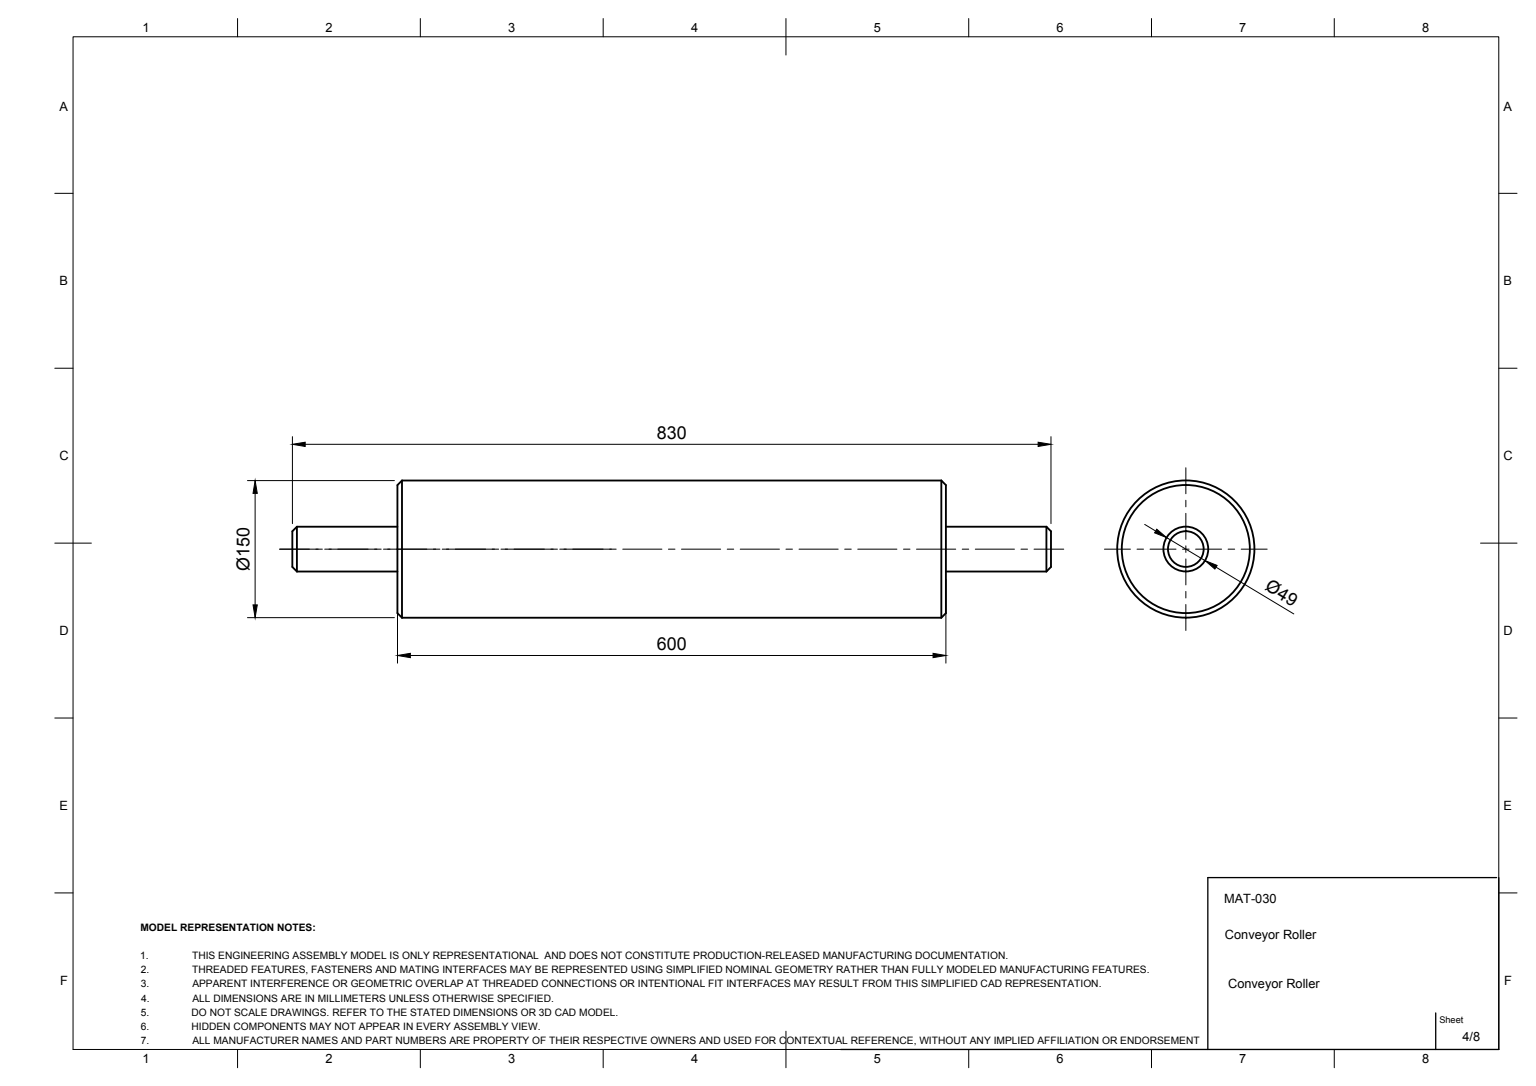
ISO-10303-21;
HEADER;
/* Generated by software containing ST-Developer
 * from STEP Tools, Inc. (www.steptools.com) 
 */

FILE_DESCRIPTION(
/* description */ ('STEP AP214'),
/* implementation_level */ '2;1');

FILE_NAME(
/* name */ 'Conveyor Roller.step',
/* time_stamp */ '2026-11-14T06:43:04-08:00',
/* author */ (''),
/* organization */ (''),
/* preprocessor_version */ 'ST-DEVELOPER v20.2',
/* originating_system */ 'Autodesk Translation Framework v15.17.0.0',
/* authorisation */ '');

FILE_SCHEMA (('AUTOMOTIVE_DESIGN { 1 0 10303 214 3 1 1 }'));
ENDSEC;

DATA;
#10=MECHANICAL_DESIGN_GEOMETRIC_PRESENTATION_REPRESENTATION('',(#205),#5658);
#107=CONICAL_SURFACE('',#3433,70.0000000000001,0.785398163397444);
#108=CONICAL_SURFACE('',#3437,19.5,0.785398163397451);
#109=CONICAL_SURFACE('',#3441,24.5,0.78539816339745);
#110=CONICAL_SURFACE('',#3444,75.,0.785398163397444);
#183=SHAPE_REPRESENTATION_RELATIONSHIP('SRR','None',#5713,#194);
#194=ADVANCED_BREP_SHAPE_REPRESENTATION('',(#216),#5654);
#205=STYLED_ITEM('',(#5773),#216);
#216=MANIFOLD_SOLID_BREP('Body1',#3067);
#262=CYLINDRICAL_SURFACE('',#3447,75.);
#263=CYLINDRICAL_SURFACE('',#3448,24.5);
#264=CYLINDRICAL_SURFACE('',#3450,24.5);
#329=FACE_BOUND('',#711,.T.);
#330=FACE_BOUND('',#713,.T.);
#462=FACE_OUTER_BOUND('',#702,.T.);
#463=FACE_OUTER_BOUND('',#703,.T.);
#464=FACE_OUTER_BOUND('',#704,.T.);
#465=FACE_OUTER_BOUND('',#705,.T.);
#466=FACE_OUTER_BOUND('',#706,.T.);
#467=FACE_OUTER_BOUND('',#707,.T.);
#468=FACE_OUTER_BOUND('',#708,.T.);
#469=FACE_OUTER_BOUND('',#709,.T.);
#470=FACE_OUTER_BOUND('',#710,.T.);
#471=FACE_OUTER_BOUND('',#712,.T.);
#472=FACE_OUTER_BOUND('',#714,.T.);
#702=EDGE_LOOP('',(#2556,#2557,#2558,#2559,#2560));
#703=EDGE_LOOP('',(#2561,#2562,#2563,#2564,#2565));
#704=EDGE_LOOP('',(#2566,#2567,#2568,#2569));
#705=EDGE_LOOP('',(#2570,#2571,#2572,#2573));
#706=EDGE_LOOP('',(#2574,#2575,#2576,#2577,#2578));
#707=EDGE_LOOP('',(#2579,#2580,#2581,#2582));
#708=EDGE_LOOP('',(#2583,#2584,#2585,#2586,#2587));
#709=EDGE_LOOP('',(#2588));
#710=EDGE_LOOP('',(#2589));
#711=EDGE_LOOP('',(#2590));
#712=EDGE_LOOP('',(#2591));
#713=EDGE_LOOP('',(#2592));
#714=EDGE_LOOP('',(#2593));
#896=LINE('',#5374,#1092);
#897=LINE('',#5382,#1093);
#898=LINE('',#5388,#1094);
#899=LINE('',#5394,#1095);
#900=LINE('',#5397,#1096);
#901=LINE('',#5401,#1097);
#902=LINE('',#5404,#1098);
#1092=VECTOR('',#4174,70.0000000000001);
#1093=VECTOR('',#4183,19.5);
#1094=VECTOR('',#4190,24.5);
#1095=VECTOR('',#4197,75.);
#1096=VECTOR('',#4202,75.);
#1097=VECTOR('',#4207,24.5);
#1098=VECTOR('',#4210,24.5);
#1266=CIRCLE('',#3434,75.);
#1267=CIRCLE('',#3435,75.);
#1268=CIRCLE('',#3436,70.0000000000001);
#1269=CIRCLE('',#3438,24.5);
#1270=CIRCLE('',#3439,24.5);
#1271=CIRCLE('',#3440,19.5);
#1272=CIRCLE('',#3442,24.5);
#1273=CIRCLE('',#3443,19.5);
#1274=CIRCLE('',#3445,75.);
#1275=CIRCLE('',#3446,70.);
#1276=CIRCLE('',#3449,24.5);
#1277=CIRCLE('',#3451,24.5);
#1499=VERTEX_POINT('',#5369);
#1500=VERTEX_POINT('',#5370);
#1501=VERTEX_POINT('',#5373);
#1502=VERTEX_POINT('',#5377);
#1503=VERTEX_POINT('',#5378);
#1504=VERTEX_POINT('',#5381);
#1505=VERTEX_POINT('',#5385);
#1506=VERTEX_POINT('',#5387);
#1507=VERTEX_POINT('',#5391);
#1508=VERTEX_POINT('',#5393);
#1509=VERTEX_POINT('',#5399);
#1510=VERTEX_POINT('',#5403);
#1861=EDGE_CURVE('',#1499,#1500,#1266,.T.);
#1862=EDGE_CURVE('',#1500,#1499,#1267,.T.);
#1863=EDGE_CURVE('',#1500,#1501,#896,.T.);
#1864=EDGE_CURVE('',#1501,#1501,#1268,.T.);
#1865=EDGE_CURVE('',#1502,#1503,#1269,.T.);
#1866=EDGE_CURVE('',#1503,#1502,#1270,.T.);
#1867=EDGE_CURVE('',#1503,#1504,#897,.T.);
#1868=EDGE_CURVE('',#1504,#1504,#1271,.T.);
#1869=EDGE_CURVE('',#1505,#1505,#1272,.T.);
#1870=EDGE_CURVE('',#1505,#1506,#898,.T.);
#1871=EDGE_CURVE('',#1506,#1506,#1273,.T.);
#1872=EDGE_CURVE('',#1507,#1507,#1274,.T.);
#1873=EDGE_CURVE('',#1507,#1508,#899,.T.);
#1874=EDGE_CURVE('',#1508,#1508,#1275,.T.);
#1875=EDGE_CURVE('',#1499,#1507,#900,.T.);
#1876=EDGE_CURVE('',#1509,#1509,#1276,.T.);
#1877=EDGE_CURVE('',#1509,#1505,#901,.T.);
#1878=EDGE_CURVE('',#1502,#1510,#902,.T.);
#1879=EDGE_CURVE('',#1510,#1510,#1277,.T.);
#2556=ORIENTED_EDGE('',*,*,#1861,.F.);
#2557=ORIENTED_EDGE('',*,*,#1862,.F.);
#2558=ORIENTED_EDGE('',*,*,#1863,.T.);
#2559=ORIENTED_EDGE('',*,*,#1864,.F.);
#2560=ORIENTED_EDGE('',*,*,#1863,.F.);
#2561=ORIENTED_EDGE('',*,*,#1865,.F.);
#2562=ORIENTED_EDGE('',*,*,#1866,.F.);
#2563=ORIENTED_EDGE('',*,*,#1867,.T.);
#2564=ORIENTED_EDGE('',*,*,#1868,.F.);
#2565=ORIENTED_EDGE('',*,*,#1867,.F.);
#2566=ORIENTED_EDGE('',*,*,#1869,.F.);
#2567=ORIENTED_EDGE('',*,*,#1870,.T.);
#2568=ORIENTED_EDGE('',*,*,#1871,.F.);
#2569=ORIENTED_EDGE('',*,*,#1870,.F.);
#2570=ORIENTED_EDGE('',*,*,#1872,.F.);
#2571=ORIENTED_EDGE('',*,*,#1873,.T.);
#2572=ORIENTED_EDGE('',*,*,#1874,.F.);
#2573=ORIENTED_EDGE('',*,*,#1873,.F.);
#2574=ORIENTED_EDGE('',*,*,#1861,.T.);
#2575=ORIENTED_EDGE('',*,*,#1862,.T.);
#2576=ORIENTED_EDGE('',*,*,#1875,.T.);
#2577=ORIENTED_EDGE('',*,*,#1872,.T.);
#2578=ORIENTED_EDGE('',*,*,#1875,.F.);
#2579=ORIENTED_EDGE('',*,*,#1876,.F.);
#2580=ORIENTED_EDGE('',*,*,#1877,.T.);
#2581=ORIENTED_EDGE('',*,*,#1869,.T.);
#2582=ORIENTED_EDGE('',*,*,#1877,.F.);
#2583=ORIENTED_EDGE('',*,*,#1865,.T.);
#2584=ORIENTED_EDGE('',*,*,#1866,.T.);
#2585=ORIENTED_EDGE('',*,*,#1878,.T.);
#2586=ORIENTED_EDGE('',*,*,#1879,.T.);
#2587=ORIENTED_EDGE('',*,*,#1878,.F.);
#2588=ORIENTED_EDGE('',*,*,#1871,.T.);
#2589=ORIENTED_EDGE('',*,*,#1874,.T.);
#2590=ORIENTED_EDGE('',*,*,#1876,.T.);
#2591=ORIENTED_EDGE('',*,*,#1864,.T.);
#2592=ORIENTED_EDGE('',*,*,#1879,.F.);
#2593=ORIENTED_EDGE('',*,*,#1868,.T.);
#2842=PLANE('',#3452);
#2843=PLANE('',#3453);
#2844=PLANE('',#3454);
#2845=PLANE('',#3455);
#3003=ADVANCED_FACE('',(#462),#107,.T.);
#3004=ADVANCED_FACE('',(#463),#108,.T.);
#3005=ADVANCED_FACE('',(#464),#109,.T.);
#3006=ADVANCED_FACE('',(#465),#110,.T.);
#3007=ADVANCED_FACE('',(#466),#262,.T.);
#3008=ADVANCED_FACE('',(#467),#263,.T.);
#3009=ADVANCED_FACE('',(#468),#264,.T.);
#3010=ADVANCED_FACE('',(#469),#2842,.T.);
#3011=ADVANCED_FACE('',(#470,#329),#2843,.T.);
#3012=ADVANCED_FACE('',(#471,#330),#2844,.F.);
#3013=ADVANCED_FACE('',(#472),#2845,.F.);
#3067=CLOSED_SHELL('',(#3003,#3004,#3005,#3006,#3007,#3008,#3009,#3010,
#3011,#3012,#3013));
#3432=AXIS2_PLACEMENT_3D('',#5367,#4166,#4167);
#3433=AXIS2_PLACEMENT_3D('',#5368,#4168,#4169);
#3434=AXIS2_PLACEMENT_3D('',#5371,#4170,#4171);
#3435=AXIS2_PLACEMENT_3D('',#5372,#4172,#4173);
#3436=AXIS2_PLACEMENT_3D('',#5375,#4175,#4176);
#3437=AXIS2_PLACEMENT_3D('',#5376,#4177,#4178);
#3438=AXIS2_PLACEMENT_3D('',#5379,#4179,#4180);
#3439=AXIS2_PLACEMENT_3D('',#5380,#4181,#4182);
#3440=AXIS2_PLACEMENT_3D('',#5383,#4184,#4185);
#3441=AXIS2_PLACEMENT_3D('',#5384,#4186,#4187);
#3442=AXIS2_PLACEMENT_3D('',#5386,#4188,#4189);
#3443=AXIS2_PLACEMENT_3D('',#5389,#4191,#4192);
#3444=AXIS2_PLACEMENT_3D('',#5390,#4193,#4194);
#3445=AXIS2_PLACEMENT_3D('',#5392,#4195,#4196);
#3446=AXIS2_PLACEMENT_3D('',#5395,#4198,#4199);
#3447=AXIS2_PLACEMENT_3D('',#5396,#4200,#4201);
#3448=AXIS2_PLACEMENT_3D('',#5398,#4203,#4204);
#3449=AXIS2_PLACEMENT_3D('',#5400,#4205,#4206);
#3450=AXIS2_PLACEMENT_3D('',#5402,#4208,#4209);
#3451=AXIS2_PLACEMENT_3D('',#5405,#4211,#4212);
#3452=AXIS2_PLACEMENT_3D('',#5406,#4213,#4214);
#3453=AXIS2_PLACEMENT_3D('',#5407,#4215,#4216);
#3454=AXIS2_PLACEMENT_3D('',#5408,#4217,#4218);
#3455=AXIS2_PLACEMENT_3D('',#5409,#4219,#4220);
#4166=DIRECTION('axis',(0.,0.,1.));
#4167=DIRECTION('refdir',(1.,0.,0.));
#4168=DIRECTION('center_axis',(0.,-1.,0.));
#4169=DIRECTION('ref_axis',(0.,0.,-1.));
#4170=DIRECTION('center_axis',(0.,-1.,0.));
#4171=DIRECTION('ref_axis',(0.,0.,-1.));
#4172=DIRECTION('center_axis',(0.,-1.,0.));
#4173=DIRECTION('ref_axis',(0.,0.,-1.));
#4174=DIRECTION('',(8.6595605623549E-17,0.70710678118655,-0.707106781186544));
#4175=DIRECTION('center_axis',(0.,1.,0.));
#4176=DIRECTION('ref_axis',(0.,0.,-1.));
#4177=DIRECTION('center_axis',(0.,-1.,0.));
#4178=DIRECTION('ref_axis',(0.,0.,-1.));
#4179=DIRECTION('center_axis',(0.,-1.,0.));
#4180=DIRECTION('ref_axis',(0.,0.,-1.));
#4181=DIRECTION('center_axis',(0.,-1.,0.));
#4182=DIRECTION('ref_axis',(0.,0.,-1.));
#4183=DIRECTION('',(8.65956056235496E-17,0.707106781186546,-0.707106781186549));
#4184=DIRECTION('center_axis',(0.,1.,0.));
#4185=DIRECTION('ref_axis',(0.,0.,-1.));
#4186=DIRECTION('center_axis',(0.,1.,0.));
#4187=DIRECTION('ref_axis',(0.,0.,1.));
#4188=DIRECTION('center_axis',(0.,1.,0.));
#4189=DIRECTION('ref_axis',(0.,0.,-1.));
#4190=DIRECTION('',(8.65956056235495E-17,-0.707106781186546,0.707106781186549));
#4191=DIRECTION('center_axis',(0.,-1.,0.));
#4192=DIRECTION('ref_axis',(0.,0.,-1.));
#4193=DIRECTION('center_axis',(0.,1.,0.));
#4194=DIRECTION('ref_axis',(0.,0.,1.));
#4195=DIRECTION('center_axis',(0.,1.,0.));
#4196=DIRECTION('ref_axis',(0.,0.,-1.));
#4197=DIRECTION('',(8.6595605623549E-17,-0.70710678118655,0.707106781186544));
#4198=DIRECTION('center_axis',(0.,-1.,0.));
#4199=DIRECTION('ref_axis',(0.,0.,-1.));
#4200=DIRECTION('center_axis',(0.,1.,0.));
#4201=DIRECTION('ref_axis',(0.,0.,1.));
#4202=DIRECTION('',(0.,-1.,0.));
#4203=DIRECTION('center_axis',(0.,1.,0.));
#4204=DIRECTION('ref_axis',(0.,0.,1.));
#4205=DIRECTION('center_axis',(0.,1.,0.));
#4206=DIRECTION('ref_axis',(0.,0.,1.));
#4207=DIRECTION('',(0.,-1.,0.));
#4208=DIRECTION('center_axis',(0.,1.,0.));
#4209=DIRECTION('ref_axis',(0.,0.,1.));
#4210=DIRECTION('',(0.,-1.,0.));
#4211=DIRECTION('center_axis',(0.,1.,0.));
#4212=DIRECTION('ref_axis',(0.,0.,1.));
#4213=DIRECTION('center_axis',(0.,-1.,0.));
#4214=DIRECTION('ref_axis',(0.,0.,-1.));
#4215=DIRECTION('center_axis',(0.,-1.,0.));
#4216=DIRECTION('ref_axis',(0.,0.,-1.));
#4217=DIRECTION('center_axis',(0.,-1.,0.));
#4218=DIRECTION('ref_axis',(0.,0.,-1.));
#4219=DIRECTION('center_axis',(0.,-1.,0.));
#4220=DIRECTION('ref_axis',(0.,0.,-1.));
#5367=CARTESIAN_POINT('',(0.,0.,0.));
#5368=CARTESIAN_POINT('Origin',(0.,300.,-2.77555756156289E-14));
#5369=CARTESIAN_POINT('',(9.18485099360515E-15,295.,-75.0000000000001));
#5370=CARTESIAN_POINT('',(-9.18485099360515E-15,295.,75.));
#5371=CARTESIAN_POINT('Origin',(0.,295.,-2.77555756156289E-14));
#5372=CARTESIAN_POINT('Origin',(0.,295.,-2.77555756156289E-14));
#5373=CARTESIAN_POINT('',(-8.57252759403148E-15,300.,70.));
#5374=CARTESIAN_POINT('',(-8.57252759403148E-15,300.,70.));
#5375=CARTESIAN_POINT('Origin',(0.,300.,-2.77555756156289E-14));
#5376=CARTESIAN_POINT('Origin',(0.,415.,-2.77555756156289E-14));
#5377=CARTESIAN_POINT('',(3.00038465791101E-15,410.,-24.5));
#5378=CARTESIAN_POINT('',(-3.00038465791101E-15,410.,24.5));
#5379=CARTESIAN_POINT('Origin',(0.,410.,-2.77555756156289E-14));
#5380=CARTESIAN_POINT('Origin',(0.,410.,-2.77555756156289E-14));
#5381=CARTESIAN_POINT('',(-2.38806125833733E-15,415.,19.4999999999999));
#5382=CARTESIAN_POINT('',(-2.38806125833733E-15,415.,19.4999999999999));
#5383=CARTESIAN_POINT('Origin',(0.,415.,-2.77555756156289E-14));
#5384=CARTESIAN_POINT('Origin',(0.,-410.,-2.77555756156289E-14));
#5385=CARTESIAN_POINT('',(-3.00038465791101E-15,-410.,-24.5));
#5386=CARTESIAN_POINT('Origin',(0.,-410.,-2.77555756156289E-14));
#5387=CARTESIAN_POINT('',(-2.38806125833733E-15,-415.,-19.5));
#5388=CARTESIAN_POINT('',(-3.00038465791101E-15,-410.,-24.5));
#5389=CARTESIAN_POINT('Origin',(0.,-415.,-2.77555756156289E-14));
#5390=CARTESIAN_POINT('Origin',(0.,-295.,-2.77555756156289E-14));
#5391=CARTESIAN_POINT('',(-9.18485099360515E-15,-295.,-75.0000000000001));
#5392=CARTESIAN_POINT('Origin',(0.,-295.,-2.77555756156289E-14));
#5393=CARTESIAN_POINT('',(-8.57252759403147E-15,-300.,-70.));
#5394=CARTESIAN_POINT('',(-9.18485099360515E-15,-295.,-75.0000000000001));
#5395=CARTESIAN_POINT('Origin',(0.,-300.,-2.77555756156289E-14));
#5396=CARTESIAN_POINT('Origin',(0.,-300.,-2.77555756156289E-14));
#5397=CARTESIAN_POINT('',(-9.18485099360515E-15,-300.,-75.0000000000001));
#5398=CARTESIAN_POINT('Origin',(0.,-300.,-2.77555756156289E-14));
#5399=CARTESIAN_POINT('',(-3.00038465791101E-15,-300.,-24.5));
#5400=CARTESIAN_POINT('Origin',(0.,-300.,-2.77555756156289E-14));
#5401=CARTESIAN_POINT('',(-3.00038465791101E-15,-300.,-24.5));
#5402=CARTESIAN_POINT('Origin',(0.,-300.,-2.77555756156289E-14));
#5403=CARTESIAN_POINT('',(-3.00038465791101E-15,300.,-24.5));
#5404=CARTESIAN_POINT('',(-3.00038465791101E-15,-300.,-24.5));
#5405=CARTESIAN_POINT('Origin',(0.,300.,-2.77555756156289E-14));
#5406=CARTESIAN_POINT('Origin',(0.,-415.,0.));
#5407=CARTESIAN_POINT('Origin',(0.,-300.,0.));
#5408=CARTESIAN_POINT('Origin',(0.,300.,0.));
#5409=CARTESIAN_POINT('Origin',(0.,415.,0.));
#5641=UNCERTAINTY_MEASURE_WITH_UNIT(LENGTH_MEASURE(0.01),#5659,
'DISTANCE_ACCURACY_VALUE',
'Maximum model space distance between geometric entities at asserted c
onnectivities');
#5645=UNCERTAINTY_MEASURE_WITH_UNIT(LENGTH_MEASURE(0.01),#5659,
'DISTANCE_ACCURACY_VALUE',
'Maximum model space distance between geometric entities at asserted c
onnectivities');
#5654=(
GEOMETRIC_REPRESENTATION_CONTEXT(3)
GLOBAL_UNCERTAINTY_ASSIGNED_CONTEXT((#5641))
GLOBAL_UNIT_ASSIGNED_CONTEXT((#5659,#5661,#5662))
REPRESENTATION_CONTEXT('','3D')
);
#5658=(
GEOMETRIC_REPRESENTATION_CONTEXT(3)
GLOBAL_UNCERTAINTY_ASSIGNED_CONTEXT((#5645))
GLOBAL_UNIT_ASSIGNED_CONTEXT((#5659,#5661,#5662))
REPRESENTATION_CONTEXT('','3D')
);
#5659=(
LENGTH_UNIT()
NAMED_UNIT(*)
SI_UNIT(.MILLI.,.METRE.)
);
#5661=(
NAMED_UNIT(*)
PLANE_ANGLE_UNIT()
SI_UNIT($,.RADIAN.)
);
#5662=(
NAMED_UNIT(*)
SI_UNIT($,.STERADIAN.)
SOLID_ANGLE_UNIT()
);
#5671=SHAPE_DEFINITION_REPRESENTATION(#5683,#5713);
#5683=PRODUCT_DEFINITION_SHAPE('',$,#5726);
#5713=SHAPE_REPRESENTATION('',(#3432),#5654);
#5717=PRODUCT_DEFINITION_CONTEXT('part definition',#5755,'design');
#5726=PRODUCT_DEFINITION('Conveyor Roller','Conveyor Roller',#5738,#5717);
#5738=PRODUCT_DEFINITION_FORMATION('',$,#5765);
#5755=APPLICATION_CONTEXT(
'Core Data for Automotive Mechanical Design Process');
#5756=PRODUCT_CONTEXT('part definition',#5755,'mechanical');
#5765=PRODUCT('Conveyor Roller','Conveyor Roller',$,(#5756));
#5773=PRESENTATION_STYLE_ASSIGNMENT((#5778));
#5778=SURFACE_STYLE_USAGE(.BOTH.,#5783);
#5783=SURFACE_SIDE_STYLE('',(#5788));
#5788=SURFACE_STYLE_FILL_AREA(#5793);
#5793=FILL_AREA_STYLE('Opaque(61,176,222)',(#5798));
#5798=FILL_AREA_STYLE_COLOUR('Opaque(61,176,222)',#5803);
#5803=COLOUR_RGB('Opaque(61,176,222)',0.23921568627451,0.690196078431373,
0.870588235294118);
ENDSEC;
END-ISO-10303-21;
